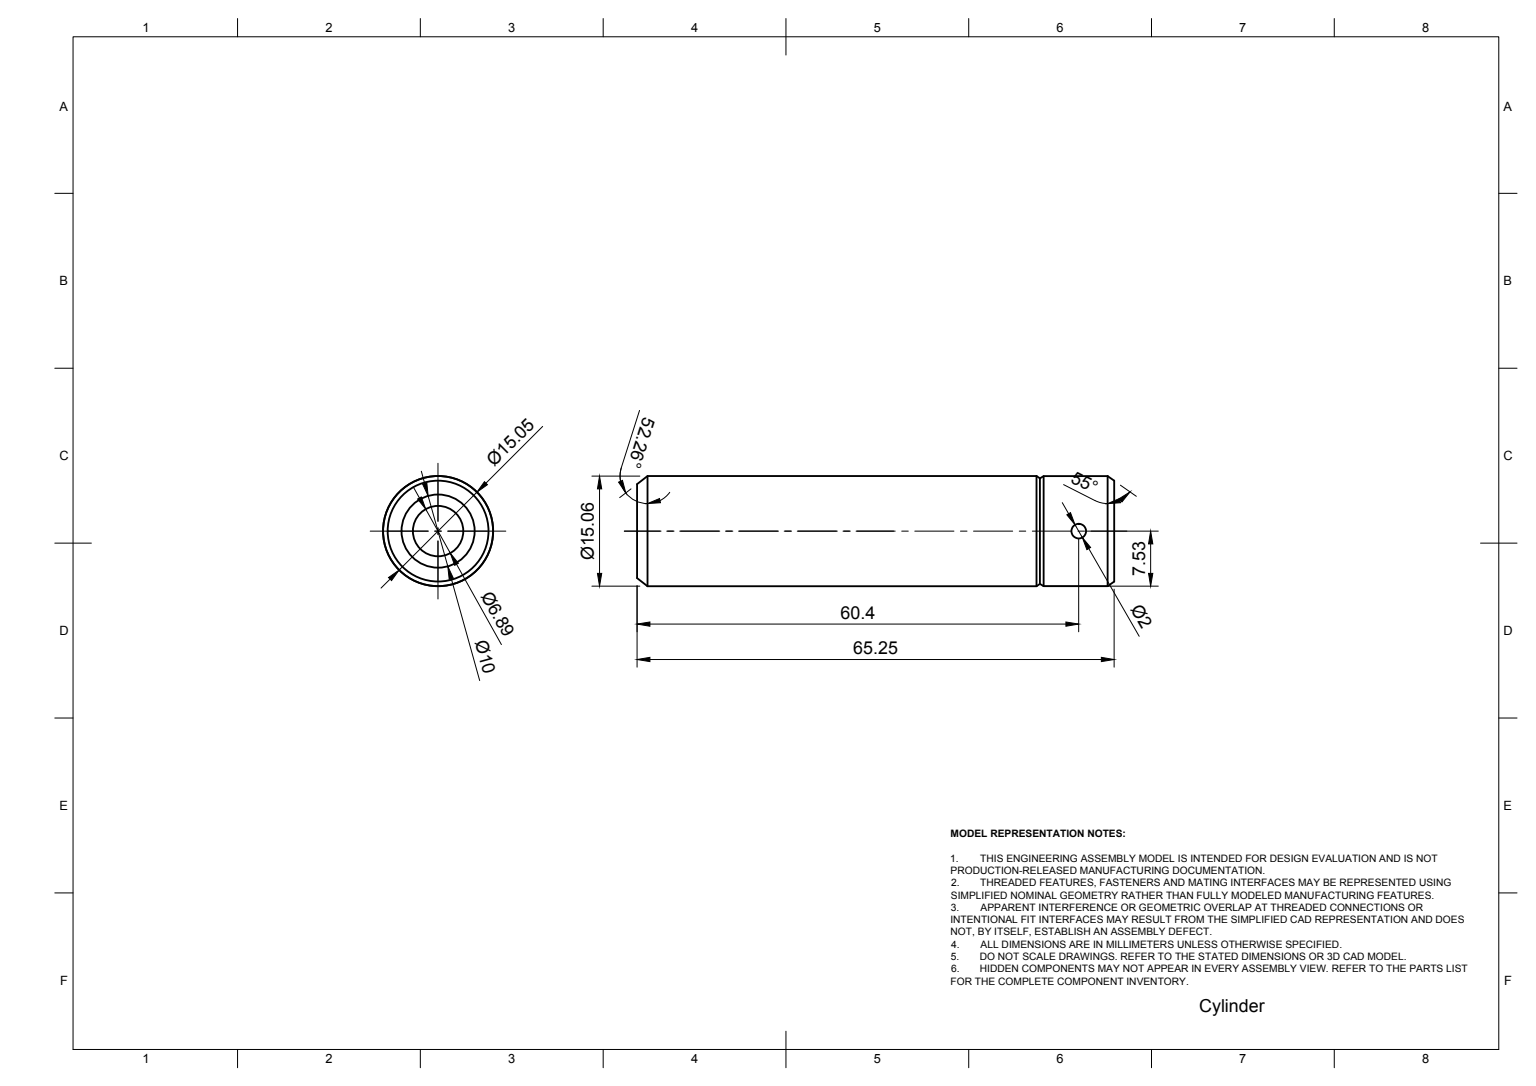
ISO-10303-21;
HEADER;
/* Generated by software containing ST-Developer
 * from STEP Tools, Inc. (www.steptools.com) 
 */

FILE_DESCRIPTION(
/* description */ (''),
/* implementation_level */ '2;1');

FILE_NAME(
/* name */ 'Cylinder.step',
/* time_stamp */ '2026-10-06T13:05:37-07:00',
/* author */ (''),
/* organization */ (''),
/* preprocessor_version */ 'ST-DEVELOPER v20.2',
/* originating_system */ 'Autodesk Translation Framework v15.15.0.0',
/* authorisation */ '');

FILE_SCHEMA (('AUTOMOTIVE_DESIGN { 1 0 10303 214 3 1 1 }'));
ENDSEC;

DATA;
#10=MECHANICAL_DESIGN_GEOMETRIC_PRESENTATION_REPRESENTATION('',(#136),#28055);
#116=SHAPE_REPRESENTATION_RELATIONSHIP('SRR','None',#28093,#126);
#126=ADVANCED_BREP_SHAPE_REPRESENTATION('',(#146),#28045);
#136=STYLED_ITEM('',(#28152),#146);
#146=MANIFOLD_SOLID_BREP('Body1',#3677);
#155=CONICAL_SURFACE('',#3808,7.20746054905241,0.610790367386849);
#156=CONICAL_SURFACE('',#3813,7.36529369971832,0.557210682142491);
#157=CONICAL_SURFACE('',#3815,7.36790580323689,0.610790367386849);
#158=CONICAL_SURFACE('',#3819,6.97561584944256,0.658634244892553);
#159=CONICAL_SURFACE('',#3821,6.41628586403442,0.000295609290232646);
#160=CONICAL_SURFACE('',#3825,6.40906719549494,0.00029560929023293);
#161=CONICAL_SURFACE('',#3833,6.40820475053297,0.000295609290233083);
#162=CONICAL_SURFACE('',#3837,6.40732538114918,0.000295609290232334);
#163=CONICAL_SURFACE('',#3841,6.40667124022599,0.000295609290231853);
#173=FACE_BOUND('',#588,.T.);
#174=FACE_BOUND('',#591,.T.);
#175=FACE_BOUND('',#600,.T.);
#176=FACE_BOUND('',#603,.T.);
#177=FACE_BOUND('',#610,.T.);
#178=FACE_BOUND('',#613,.T.);
#179=FACE_BOUND('',#615,.T.);
#180=FACE_BOUND('',#617,.T.);
#203=PLANE('',#3806);
#204=PLANE('',#3827);
#205=PLANE('',#3831);
#206=PLANE('',#3843);
#207=PLANE('',#3847);
#208=PLANE('',#3850);
#256=CIRCLE('',#3804,5.);
#257=CIRCLE('',#3805,5.);
#258=CIRCLE('',#3807,3.44589712386029);
#259=CIRCLE('',#3809,7.52312685038423);
#260=CIRCLE('',#3810,6.89179424772059);
#261=CIRCLE('',#3812,7.52312685038423);
#262=CIRCLE('',#3814,7.20746054905241);
#263=CIRCLE('',#3816,7.52835105742136);
#264=CIRCLE('',#3818,7.52835105742136);
#265=CIRCLE('',#3820,6.42288064146375);
#266=CIRCLE('',#3822,6.40969108660508);
#267=CIRCLE('',#3824,6.40969108660508);
#268=CIRCLE('',#3826,6.40881029802658);
#269=CIRCLE('',#3828,6.41550316824698);
#270=CIRCLE('',#3830,6.41550316824698);
#271=CIRCLE('',#3832,6.40853872070288);
#272=CIRCLE('',#3834,6.40787078036307);
#273=CIRCLE('',#3836,6.40787078036307);
#274=CIRCLE('',#3838,6.40706623219228);
#275=CIRCLE('',#3840,6.40706623219228);
#276=CIRCLE('',#3842,6.4065967297173);
#277=CIRCLE('',#3844,4.66385643997278);
#278=CIRCLE('',#3846,4.66385643997278);
#279=CIRCLE('',#3848,3.44589712386029);
#379=FACE_OUTER_BOUND('',#585,.T.);
#380=FACE_OUTER_BOUND('',#586,.T.);
#381=FACE_OUTER_BOUND('',#587,.T.);
#382=FACE_OUTER_BOUND('',#589,.T.);
#383=FACE_OUTER_BOUND('',#590,.T.);
#384=FACE_OUTER_BOUND('',#592,.T.);
#385=FACE_OUTER_BOUND('',#593,.T.);
#386=FACE_OUTER_BOUND('',#594,.T.);
#387=FACE_OUTER_BOUND('',#595,.T.);
#388=FACE_OUTER_BOUND('',#596,.T.);
#389=FACE_OUTER_BOUND('',#597,.T.);
#390=FACE_OUTER_BOUND('',#598,.T.);
#391=FACE_OUTER_BOUND('',#599,.T.);
#392=FACE_OUTER_BOUND('',#601,.T.);
#393=FACE_OUTER_BOUND('',#602,.T.);
#394=FACE_OUTER_BOUND('',#604,.T.);
#395=FACE_OUTER_BOUND('',#605,.T.);
#396=FACE_OUTER_BOUND('',#606,.T.);
#397=FACE_OUTER_BOUND('',#607,.T.);
#398=FACE_OUTER_BOUND('',#608,.T.);
#399=FACE_OUTER_BOUND('',#609,.T.);
#400=FACE_OUTER_BOUND('',#611,.T.);
#401=FACE_OUTER_BOUND('',#612,.T.);
#402=FACE_OUTER_BOUND('',#614,.T.);
#403=FACE_OUTER_BOUND('',#616,.T.);
#585=EDGE_LOOP('',(#2310,#2311,#2312,#2313,#2314,#2315));
#586=EDGE_LOOP('',(#2316,#2317,#2318,#2319));
#587=EDGE_LOOP('',(#2320));
#588=EDGE_LOOP('',(#2321));
#589=EDGE_LOOP('',(#2322,#2323,#2324,#2325));
#590=EDGE_LOOP('',(#2326,#2327,#2328,#2329));
#591=EDGE_LOOP('',(#2330,#2331));
#592=EDGE_LOOP('',(#2332,#2333,#2334,#2335));
#593=EDGE_LOOP('',(#2336,#2337,#2338,#2339));
#594=EDGE_LOOP('',(#2340,#2341,#2342,#2343));
#595=EDGE_LOOP('',(#2344,#2345,#2346,#2347));
#596=EDGE_LOOP('',(#2348,#2349,#2350,#2351));
#597=EDGE_LOOP('',(#2352,#2353,#2354,#2355));
#598=EDGE_LOOP('',(#2356,#2357,#2358,#2359));
#599=EDGE_LOOP('',(#2360));
#600=EDGE_LOOP('',(#2361));
#601=EDGE_LOOP('',(#2362,#2363,#2364,#2365));
#602=EDGE_LOOP('',(#2366));
#603=EDGE_LOOP('',(#2367));
#604=EDGE_LOOP('',(#2368,#2369,#2370,#2371));
#605=EDGE_LOOP('',(#2372,#2373,#2374,#2375));
#606=EDGE_LOOP('',(#2376,#2377,#2378,#2379));
#607=EDGE_LOOP('',(#2380,#2381,#2382,#2383));
#608=EDGE_LOOP('',(#2384,#2385,#2386,#2387));
#609=EDGE_LOOP('',(#2388));
#610=EDGE_LOOP('',(#2389));
#611=EDGE_LOOP('',(#2390,#2391,#2392,#2393));
#612=EDGE_LOOP('',(#2394));
#613=EDGE_LOOP('',(#2395));
#614=EDGE_LOOP('',(#2396,#2397,#2398,#2399));
#615=EDGE_LOOP('',(#2400,#2401));
#616=EDGE_LOOP('',(#2402));
#617=EDGE_LOOP('',(#2403));
#821=LINE('',#4942,#979);
#822=LINE('',#4984,#980);
#823=LINE('',#4993,#981);
#824=LINE('',#4998,#982);
#825=LINE('',#5001,#983);
#826=LINE('',#5006,#984);
#827=LINE('',#5010,#985);
#828=LINE('',#5013,#986);
#829=LINE('',#5018,#987);
#830=LINE('',#5022,#988);
#831=LINE('',#5026,#989);
#832=LINE('',#5033,#990);
#833=LINE('',#5040,#991);
#834=LINE('',#5044,#992);
#835=LINE('',#5048,#993);
#836=LINE('',#5052,#994);
#837=LINE('',#5056,#995);
#838=LINE('',#5063,#996);
#839=LINE('',#5068,#997);
#979=VECTOR('',#4120,0.999999999999999);
#980=VECTOR('',#4125,5.);
#981=VECTOR('',#4136,7.20746054905241);
#982=VECTOR('',#4143,7.52312685038423);
#983=VECTOR('',#4146,7.36529369971832);
#984=VECTOR('',#4153,7.36790580323689);
#985=VECTOR('',#4158,7.52835105742136);
#986=VECTOR('',#4161,6.97561584944256);
#987=VECTOR('',#4168,6.41628586403442);
#988=VECTOR('',#4173,6.40969108660508);
#989=VECTOR('',#4178,6.40906719549494);
#990=VECTOR('',#4187,6.41550316824698);
#991=VECTOR('',#4196,6.40820475053297);
#992=VECTOR('',#4201,6.40787078036307);
#993=VECTOR('',#4206,6.40732538114918);
#994=VECTOR('',#4211,6.40706623219228);
#995=VECTOR('',#4216,6.40667124022599);
#996=VECTOR('',#4225,4.66385643997278);
#997=VECTOR('',#4232,3.44589712386029);
#1137=B_SPLINE_CURVE_WITH_KNOTS('',3,(#4905,#4906,#4907,#4908,#4909,#4910,
#4911,#4912,#4913,#4914,#4915,#4916,#4917,#4918,#4919,#4920,#4921,#4922,
#4923,#4924,#4925,#4926,#4927,#4928,#4929,#4930),.UNSPECIFIED.,.F.,.F.,
(4,2,2,2,2,2,2,2,2,2,2,2,4),(-0.606481282784619,-0.568571286664201,-0.530661290543783,
-0.492761126316124,-0.454860962088464,-0.416960797860805,-0.379060633633146,
-0.341150637512728,-0.30324064139231,-0.265330645271891,-0.227420649151473,
-0.189520484923814,-0.151620320696155),.UNSPECIFIED.);
#1138=B_SPLINE_CURVE_WITH_KNOTS('',3,(#4931,#4932,#4933,#4934,#4935,#4936,
#4937,#4938,#4939,#4940),.UNSPECIFIED.,.F.,.F.,(4,2,2,2,4),(-0.151620320696155,
-0.113720156468496,-0.0758199922408364,-0.0379099961204182,0.),
 .UNSPECIFIED.);
#1139=B_SPLINE_CURVE_WITH_KNOTS('',3,(#4944,#4945,#4946,#4947,#4948,#4949,
#4950,#4951,#4952,#4953),.UNSPECIFIED.,.F.,.F.,(4,2,2,2,4),(0.,0.0377168406459521,
0.0754336812919042,0.113150118256495,0.150866555221085),.UNSPECIFIED.);
#1140=B_SPLINE_CURVE_WITH_KNOTS('',3,(#4954,#4955,#4956,#4957,#4958,#4959,
#4960,#4961,#4962,#4963,#4964,#4965,#4966,#4967,#4968,#4969,#4970,#4971,
#4972,#4973,#4974,#4975,#4976,#4977,#4978,#4979),.UNSPECIFIED.,.F.,.F.,
(4,2,2,2,2,2,2,2,2,2,2,2,4),(0.150866555221085,0.188582992185676,0.226299429150267,
0.264016269796219,0.301733110442171,0.339449951088123,0.377166791734075,
0.414883228698666,0.452599665663256,0.490316102627847,0.528032539592437,
0.565749380238389,0.603466220884342),.UNSPECIFIED.);
#1394=VERTEX_POINT('',#4903);
#1395=VERTEX_POINT('',#4904);
#1396=VERTEX_POINT('',#4941);
#1397=VERTEX_POINT('',#4943);
#1398=VERTEX_POINT('',#4981);
#1399=VERTEX_POINT('',#4983);
#1400=VERTEX_POINT('',#4987);
#1401=VERTEX_POINT('',#4990);
#1402=VERTEX_POINT('',#4992);
#1403=VERTEX_POINT('',#4996);
#1404=VERTEX_POINT('',#5000);
#1405=VERTEX_POINT('',#5004);
#1406=VERTEX_POINT('',#5008);
#1407=VERTEX_POINT('',#5012);
#1408=VERTEX_POINT('',#5016);
#1409=VERTEX_POINT('',#5020);
#1410=VERTEX_POINT('',#5024);
#1411=VERTEX_POINT('',#5028);
#1412=VERTEX_POINT('',#5031);
#1413=VERTEX_POINT('',#5035);
#1414=VERTEX_POINT('',#5038);
#1415=VERTEX_POINT('',#5042);
#1416=VERTEX_POINT('',#5046);
#1417=VERTEX_POINT('',#5050);
#1418=VERTEX_POINT('',#5054);
#1419=VERTEX_POINT('',#5058);
#1420=VERTEX_POINT('',#5061);
#1421=VERTEX_POINT('',#5065);
#1768=EDGE_CURVE('',#1394,#1395,#1137,.T.);
#1769=EDGE_CURVE('',#1395,#1394,#1138,.T.);
#1770=EDGE_CURVE('',#1395,#1396,#821,.T.);
#1771=EDGE_CURVE('',#1397,#1396,#1139,.T.);
#1772=EDGE_CURVE('',#1396,#1397,#1140,.T.);
#1773=EDGE_CURVE('',#1398,#1398,#256,.T.);
#1774=EDGE_CURVE('',#1398,#1399,#822,.T.);
#1775=EDGE_CURVE('',#1399,#1399,#257,.T.);
#1776=EDGE_CURVE('',#1400,#1400,#258,.T.);
#1777=EDGE_CURVE('',#1401,#1401,#259,.T.);
#1778=EDGE_CURVE('',#1401,#1402,#823,.T.);
#1779=EDGE_CURVE('',#1402,#1402,#260,.T.);
#1780=EDGE_CURVE('',#1403,#1403,#261,.T.);
#1781=EDGE_CURVE('',#1403,#1401,#824,.T.);
#1782=EDGE_CURVE('',#1403,#1404,#825,.T.);
#1783=EDGE_CURVE('',#1404,#1404,#262,.T.);
#1784=EDGE_CURVE('',#1405,#1405,#263,.T.);
#1785=EDGE_CURVE('',#1405,#1404,#826,.T.);
#1786=EDGE_CURVE('',#1406,#1406,#264,.T.);
#1787=EDGE_CURVE('',#1406,#1405,#827,.T.);
#1788=EDGE_CURVE('',#1406,#1407,#828,.T.);
#1789=EDGE_CURVE('',#1407,#1407,#265,.T.);
#1790=EDGE_CURVE('',#1408,#1408,#266,.T.);
#1791=EDGE_CURVE('',#1408,#1407,#829,.T.);
#1792=EDGE_CURVE('',#1409,#1409,#267,.T.);
#1793=EDGE_CURVE('',#1409,#1408,#830,.T.);
#1794=EDGE_CURVE('',#1410,#1410,#268,.T.);
#1795=EDGE_CURVE('',#1410,#1409,#831,.T.);
#1796=EDGE_CURVE('',#1411,#1411,#269,.T.);
#1797=EDGE_CURVE('',#1412,#1412,#270,.T.);
#1798=EDGE_CURVE('',#1412,#1411,#832,.T.);
#1799=EDGE_CURVE('',#1413,#1413,#271,.T.);
#1800=EDGE_CURVE('',#1414,#1414,#272,.T.);
#1801=EDGE_CURVE('',#1414,#1413,#833,.T.);
#1802=EDGE_CURVE('',#1415,#1415,#273,.T.);
#1803=EDGE_CURVE('',#1415,#1414,#834,.T.);
#1804=EDGE_CURVE('',#1416,#1416,#274,.T.);
#1805=EDGE_CURVE('',#1416,#1415,#835,.T.);
#1806=EDGE_CURVE('',#1417,#1417,#275,.T.);
#1807=EDGE_CURVE('',#1417,#1416,#836,.T.);
#1808=EDGE_CURVE('',#1418,#1418,#276,.T.);
#1809=EDGE_CURVE('',#1418,#1417,#837,.T.);
#1810=EDGE_CURVE('',#1419,#1419,#277,.T.);
#1811=EDGE_CURVE('',#1420,#1420,#278,.T.);
#1812=EDGE_CURVE('',#1420,#1419,#838,.T.);
#1813=EDGE_CURVE('',#1421,#1421,#279,.T.);
#1814=EDGE_CURVE('',#1400,#1421,#839,.T.);
#2310=ORIENTED_EDGE('',*,*,#1768,.F.);
#2311=ORIENTED_EDGE('',*,*,#1769,.F.);
#2312=ORIENTED_EDGE('',*,*,#1770,.T.);
#2313=ORIENTED_EDGE('',*,*,#1771,.F.);
#2314=ORIENTED_EDGE('',*,*,#1772,.F.);
#2315=ORIENTED_EDGE('',*,*,#1770,.F.);
#2316=ORIENTED_EDGE('',*,*,#1773,.F.);
#2317=ORIENTED_EDGE('',*,*,#1774,.T.);
#2318=ORIENTED_EDGE('',*,*,#1775,.T.);
#2319=ORIENTED_EDGE('',*,*,#1774,.F.);
#2320=ORIENTED_EDGE('',*,*,#1775,.F.);
#2321=ORIENTED_EDGE('',*,*,#1776,.T.);
#2322=ORIENTED_EDGE('',*,*,#1777,.F.);
#2323=ORIENTED_EDGE('',*,*,#1778,.T.);
#2324=ORIENTED_EDGE('',*,*,#1779,.T.);
#2325=ORIENTED_EDGE('',*,*,#1778,.F.);
#2326=ORIENTED_EDGE('',*,*,#1780,.F.);
#2327=ORIENTED_EDGE('',*,*,#1781,.T.);
#2328=ORIENTED_EDGE('',*,*,#1777,.T.);
#2329=ORIENTED_EDGE('',*,*,#1781,.F.);
#2330=ORIENTED_EDGE('',*,*,#1771,.T.);
#2331=ORIENTED_EDGE('',*,*,#1772,.T.);
#2332=ORIENTED_EDGE('',*,*,#1780,.T.);
#2333=ORIENTED_EDGE('',*,*,#1782,.T.);
#2334=ORIENTED_EDGE('',*,*,#1783,.F.);
#2335=ORIENTED_EDGE('',*,*,#1782,.F.);
#2336=ORIENTED_EDGE('',*,*,#1784,.F.);
#2337=ORIENTED_EDGE('',*,*,#1785,.T.);
#2338=ORIENTED_EDGE('',*,*,#1783,.T.);
#2339=ORIENTED_EDGE('',*,*,#1785,.F.);
#2340=ORIENTED_EDGE('',*,*,#1786,.F.);
#2341=ORIENTED_EDGE('',*,*,#1787,.T.);
#2342=ORIENTED_EDGE('',*,*,#1784,.T.);
#2343=ORIENTED_EDGE('',*,*,#1787,.F.);
#2344=ORIENTED_EDGE('',*,*,#1786,.T.);
#2345=ORIENTED_EDGE('',*,*,#1788,.T.);
#2346=ORIENTED_EDGE('',*,*,#1789,.F.);
#2347=ORIENTED_EDGE('',*,*,#1788,.F.);
#2348=ORIENTED_EDGE('',*,*,#1790,.F.);
#2349=ORIENTED_EDGE('',*,*,#1791,.T.);
#2350=ORIENTED_EDGE('',*,*,#1789,.T.);
#2351=ORIENTED_EDGE('',*,*,#1791,.F.);
#2352=ORIENTED_EDGE('',*,*,#1792,.F.);
#2353=ORIENTED_EDGE('',*,*,#1793,.T.);
#2354=ORIENTED_EDGE('',*,*,#1790,.T.);
#2355=ORIENTED_EDGE('',*,*,#1793,.F.);
#2356=ORIENTED_EDGE('',*,*,#1794,.F.);
#2357=ORIENTED_EDGE('',*,*,#1795,.T.);
#2358=ORIENTED_EDGE('',*,*,#1792,.T.);
#2359=ORIENTED_EDGE('',*,*,#1795,.F.);
#2360=ORIENTED_EDGE('',*,*,#1796,.F.);
#2361=ORIENTED_EDGE('',*,*,#1794,.T.);
#2362=ORIENTED_EDGE('',*,*,#1797,.F.);
#2363=ORIENTED_EDGE('',*,*,#1798,.T.);
#2364=ORIENTED_EDGE('',*,*,#1796,.T.);
#2365=ORIENTED_EDGE('',*,*,#1798,.F.);
#2366=ORIENTED_EDGE('',*,*,#1797,.T.);
#2367=ORIENTED_EDGE('',*,*,#1799,.F.);
#2368=ORIENTED_EDGE('',*,*,#1800,.F.);
#2369=ORIENTED_EDGE('',*,*,#1801,.T.);
#2370=ORIENTED_EDGE('',*,*,#1799,.T.);
#2371=ORIENTED_EDGE('',*,*,#1801,.F.);
#2372=ORIENTED_EDGE('',*,*,#1802,.F.);
#2373=ORIENTED_EDGE('',*,*,#1803,.T.);
#2374=ORIENTED_EDGE('',*,*,#1800,.T.);
#2375=ORIENTED_EDGE('',*,*,#1803,.F.);
#2376=ORIENTED_EDGE('',*,*,#1804,.F.);
#2377=ORIENTED_EDGE('',*,*,#1805,.T.);
#2378=ORIENTED_EDGE('',*,*,#1802,.T.);
#2379=ORIENTED_EDGE('',*,*,#1805,.F.);
#2380=ORIENTED_EDGE('',*,*,#1806,.F.);
#2381=ORIENTED_EDGE('',*,*,#1807,.T.);
#2382=ORIENTED_EDGE('',*,*,#1804,.T.);
#2383=ORIENTED_EDGE('',*,*,#1807,.F.);
#2384=ORIENTED_EDGE('',*,*,#1808,.F.);
#2385=ORIENTED_EDGE('',*,*,#1809,.T.);
#2386=ORIENTED_EDGE('',*,*,#1806,.T.);
#2387=ORIENTED_EDGE('',*,*,#1809,.F.);
#2388=ORIENTED_EDGE('',*,*,#1808,.T.);
#2389=ORIENTED_EDGE('',*,*,#1810,.F.);
#2390=ORIENTED_EDGE('',*,*,#1811,.F.);
#2391=ORIENTED_EDGE('',*,*,#1812,.T.);
#2392=ORIENTED_EDGE('',*,*,#1810,.T.);
#2393=ORIENTED_EDGE('',*,*,#1812,.F.);
#2394=ORIENTED_EDGE('',*,*,#1811,.T.);
#2395=ORIENTED_EDGE('',*,*,#1813,.F.);
#2396=ORIENTED_EDGE('',*,*,#1776,.F.);
#2397=ORIENTED_EDGE('',*,*,#1814,.T.);
#2398=ORIENTED_EDGE('',*,*,#1813,.T.);
#2399=ORIENTED_EDGE('',*,*,#1814,.F.);
#2400=ORIENTED_EDGE('',*,*,#1768,.T.);
#2401=ORIENTED_EDGE('',*,*,#1769,.T.);
#2402=ORIENTED_EDGE('',*,*,#1779,.F.);
#2403=ORIENTED_EDGE('',*,*,#1773,.T.);
#3394=CYLINDRICAL_SURFACE('',#3802,0.999999999999999);
#3395=CYLINDRICAL_SURFACE('',#3803,5.);
#3396=CYLINDRICAL_SURFACE('',#3811,7.52312685038423);
#3397=CYLINDRICAL_SURFACE('',#3817,7.52835105742136);
#3398=CYLINDRICAL_SURFACE('',#3823,6.40969108660508);
#3399=CYLINDRICAL_SURFACE('',#3829,6.41550316824698);
#3400=CYLINDRICAL_SURFACE('',#3835,6.40787078036307);
#3401=CYLINDRICAL_SURFACE('',#3839,6.40706623219228);
#3402=CYLINDRICAL_SURFACE('',#3845,4.66385643997278);
#3403=CYLINDRICAL_SURFACE('',#3849,3.44589712386029);
#3471=ADVANCED_FACE('',(#379),#3394,.F.);
#3472=ADVANCED_FACE('',(#380),#3395,.F.);
#3473=ADVANCED_FACE('',(#381,#173),#203,.T.);
#3474=ADVANCED_FACE('',(#382),#155,.T.);
#3475=ADVANCED_FACE('',(#383,#174),#3396,.T.);
#3476=ADVANCED_FACE('',(#384),#156,.T.);
#3477=ADVANCED_FACE('',(#385),#157,.T.);
#3478=ADVANCED_FACE('',(#386),#3397,.T.);
#3479=ADVANCED_FACE('',(#387),#158,.T.);
#3480=ADVANCED_FACE('',(#388),#159,.F.);
#3481=ADVANCED_FACE('',(#389),#3398,.F.);
#3482=ADVANCED_FACE('',(#390),#160,.F.);
#3483=ADVANCED_FACE('',(#391,#175),#204,.T.);
#3484=ADVANCED_FACE('',(#392),#3399,.F.);
#3485=ADVANCED_FACE('',(#393,#176),#205,.T.);
#3486=ADVANCED_FACE('',(#394),#161,.F.);
#3487=ADVANCED_FACE('',(#395),#3400,.F.);
#3488=ADVANCED_FACE('',(#396),#162,.F.);
#3489=ADVANCED_FACE('',(#397),#3401,.F.);
#3490=ADVANCED_FACE('',(#398),#163,.F.);
#3491=ADVANCED_FACE('',(#399,#177),#206,.T.);
#3492=ADVANCED_FACE('',(#400),#3402,.F.);
#3493=ADVANCED_FACE('',(#401,#178),#207,.T.);
#3494=ADVANCED_FACE('',(#402,#179),#3403,.F.);
#3495=ADVANCED_FACE('',(#403,#180),#208,.T.);
#3677=CLOSED_SHELL('',(#3471,#3472,#3473,#3474,#3475,#3476,#3477,#3478,
#3479,#3480,#3481,#3482,#3483,#3484,#3485,#3486,#3487,#3488,#3489,#3490,
#3491,#3492,#3493,#3494,#3495));
#3801=AXIS2_PLACEMENT_3D('',#4901,#4116,#4117);
#3802=AXIS2_PLACEMENT_3D('',#4902,#4118,#4119);
#3803=AXIS2_PLACEMENT_3D('',#4980,#4121,#4122);
#3804=AXIS2_PLACEMENT_3D('',#4982,#4123,#4124);
#3805=AXIS2_PLACEMENT_3D('',#4985,#4126,#4127);
#3806=AXIS2_PLACEMENT_3D('',#4986,#4128,#4129);
#3807=AXIS2_PLACEMENT_3D('',#4988,#4130,#4131);
#3808=AXIS2_PLACEMENT_3D('',#4989,#4132,#4133);
#3809=AXIS2_PLACEMENT_3D('',#4991,#4134,#4135);
#3810=AXIS2_PLACEMENT_3D('',#4994,#4137,#4138);
#3811=AXIS2_PLACEMENT_3D('',#4995,#4139,#4140);
#3812=AXIS2_PLACEMENT_3D('',#4997,#4141,#4142);
#3813=AXIS2_PLACEMENT_3D('',#4999,#4144,#4145);
#3814=AXIS2_PLACEMENT_3D('',#5002,#4147,#4148);
#3815=AXIS2_PLACEMENT_3D('',#5003,#4149,#4150);
#3816=AXIS2_PLACEMENT_3D('',#5005,#4151,#4152);
#3817=AXIS2_PLACEMENT_3D('',#5007,#4154,#4155);
#3818=AXIS2_PLACEMENT_3D('',#5009,#4156,#4157);
#3819=AXIS2_PLACEMENT_3D('',#5011,#4159,#4160);
#3820=AXIS2_PLACEMENT_3D('',#5014,#4162,#4163);
#3821=AXIS2_PLACEMENT_3D('',#5015,#4164,#4165);
#3822=AXIS2_PLACEMENT_3D('',#5017,#4166,#4167);
#3823=AXIS2_PLACEMENT_3D('',#5019,#4169,#4170);
#3824=AXIS2_PLACEMENT_3D('',#5021,#4171,#4172);
#3825=AXIS2_PLACEMENT_3D('',#5023,#4174,#4175);
#3826=AXIS2_PLACEMENT_3D('',#5025,#4176,#4177);
#3827=AXIS2_PLACEMENT_3D('',#5027,#4179,#4180);
#3828=AXIS2_PLACEMENT_3D('',#5029,#4181,#4182);
#3829=AXIS2_PLACEMENT_3D('',#5030,#4183,#4184);
#3830=AXIS2_PLACEMENT_3D('',#5032,#4185,#4186);
#3831=AXIS2_PLACEMENT_3D('',#5034,#4188,#4189);
#3832=AXIS2_PLACEMENT_3D('',#5036,#4190,#4191);
#3833=AXIS2_PLACEMENT_3D('',#5037,#4192,#4193);
#3834=AXIS2_PLACEMENT_3D('',#5039,#4194,#4195);
#3835=AXIS2_PLACEMENT_3D('',#5041,#4197,#4198);
#3836=AXIS2_PLACEMENT_3D('',#5043,#4199,#4200);
#3837=AXIS2_PLACEMENT_3D('',#5045,#4202,#4203);
#3838=AXIS2_PLACEMENT_3D('',#5047,#4204,#4205);
#3839=AXIS2_PLACEMENT_3D('',#5049,#4207,#4208);
#3840=AXIS2_PLACEMENT_3D('',#5051,#4209,#4210);
#3841=AXIS2_PLACEMENT_3D('',#5053,#4212,#4213);
#3842=AXIS2_PLACEMENT_3D('',#5055,#4214,#4215);
#3843=AXIS2_PLACEMENT_3D('',#5057,#4217,#4218);
#3844=AXIS2_PLACEMENT_3D('',#5059,#4219,#4220);
#3845=AXIS2_PLACEMENT_3D('',#5060,#4221,#4222);
#3846=AXIS2_PLACEMENT_3D('',#5062,#4223,#4224);
#3847=AXIS2_PLACEMENT_3D('',#5064,#4226,#4227);
#3848=AXIS2_PLACEMENT_3D('',#5066,#4228,#4229);
#3849=AXIS2_PLACEMENT_3D('',#5067,#4230,#4231);
#3850=AXIS2_PLACEMENT_3D('',#5069,#4233,#4234);
#4116=DIRECTION('axis',(0.,0.,1.));
#4117=DIRECTION('refdir',(1.,0.,0.));
#4118=DIRECTION('center_axis',(0.,1.,0.));
#4119=DIRECTION('ref_axis',(1.,0.,0.));
#4120=DIRECTION('',(0.,1.,0.));
#4121=DIRECTION('center_axis',(1.,0.,0.));
#4122=DIRECTION('ref_axis',(0.,-1.,0.));
#4123=DIRECTION('center_axis',(1.,0.,0.));
#4124=DIRECTION('ref_axis',(0.,-1.,0.));
#4125=DIRECTION('',(1.,0.,0.));
#4126=DIRECTION('center_axis',(1.,0.,0.));
#4127=DIRECTION('ref_axis',(0.,-1.,0.));
#4128=DIRECTION('center_axis',(-1.,0.,0.));
#4129=DIRECTION('ref_axis',(0.,-1.,0.));
#4130=DIRECTION('center_axis',(1.,0.,0.));
#4131=DIRECTION('ref_axis',(0.,0.,-1.));
#4132=DIRECTION('center_axis',(1.,0.,0.));
#4133=DIRECTION('ref_axis',(0.,0.,-1.));
#4134=DIRECTION('center_axis',(1.,0.,0.));
#4135=DIRECTION('ref_axis',(0.,0.,-1.));
#4136=DIRECTION('',(-0.819194986126072,7.02353436578877E-17,-0.573515104165448));
#4137=DIRECTION('center_axis',(1.,0.,0.));
#4138=DIRECTION('ref_axis',(0.,0.,-1.));
#4139=DIRECTION('center_axis',(1.,0.,0.));
#4140=DIRECTION('ref_axis',(0.,0.,-1.));
#4141=DIRECTION('center_axis',(1.,0.,0.));
#4142=DIRECTION('ref_axis',(0.,0.,-1.));
#4143=DIRECTION('',(-1.,0.,0.));
#4144=DIRECTION('center_axis',(-1.,0.,0.));
#4145=DIRECTION('ref_axis',(0.,0.,-1.));
#4146=DIRECTION('',(0.848733460294827,-6.47618786727041E-17,-0.528820870783264));
#4147=DIRECTION('center_axis',(1.,0.,0.));
#4148=DIRECTION('ref_axis',(0.,0.,-1.));
#4149=DIRECTION('center_axis',(1.,0.,0.));
#4150=DIRECTION('ref_axis',(0.,0.,-1.));
#4151=DIRECTION('center_axis',(1.,0.,0.));
#4152=DIRECTION('ref_axis',(0.,0.,-1.));
#4153=DIRECTION('',(-0.819194986126072,7.02353436578877E-17,-0.573515104165448));
#4154=DIRECTION('center_axis',(1.,0.,0.));
#4155=DIRECTION('ref_axis',(0.,0.,-1.));
#4156=DIRECTION('center_axis',(1.,0.,0.));
#4157=DIRECTION('ref_axis',(0.,0.,-1.));
#4158=DIRECTION('',(-1.,0.,0.));
#4159=DIRECTION('center_axis',(-1.,0.,0.));
#4160=DIRECTION('ref_axis',(0.,0.,-1.));
#4161=DIRECTION('',(0.790828861928077,-7.49529574979538E-17,-0.612037344564482));
#4162=DIRECTION('center_axis',(1.,0.,0.));
#4163=DIRECTION('ref_axis',(0.,0.,-1.));
#4164=DIRECTION('center_axis',(1.,0.,0.));
#4165=DIRECTION('ref_axis',(0.,0.,-1.));
#4166=DIRECTION('center_axis',(1.,0.,0.));
#4167=DIRECTION('ref_axis',(0.,0.,-1.));
#4168=DIRECTION('',(0.999999956307574,-3.62016965809164E-20,0.00029560928592735));
#4169=DIRECTION('center_axis',(1.,0.,0.));
#4170=DIRECTION('ref_axis',(0.,0.,-1.));
#4171=DIRECTION('center_axis',(1.,0.,0.));
#4172=DIRECTION('ref_axis',(0.,0.,-1.));
#4173=DIRECTION('',(1.,0.,0.));
#4174=DIRECTION('center_axis',(1.,0.,0.));
#4175=DIRECTION('ref_axis',(0.,0.,-1.));
#4176=DIRECTION('center_axis',(1.,0.,0.));
#4177=DIRECTION('ref_axis',(0.,0.,-1.));
#4178=DIRECTION('',(0.999999956307574,-3.62016965809512E-20,0.000295609285927634));
#4179=DIRECTION('center_axis',(-1.,0.,0.));
#4180=DIRECTION('ref_axis',(0.,0.,1.));
#4181=DIRECTION('center_axis',(1.,0.,0.));
#4182=DIRECTION('ref_axis',(0.,0.,-1.));
#4183=DIRECTION('center_axis',(1.,0.,0.));
#4184=DIRECTION('ref_axis',(0.,0.,-1.));
#4185=DIRECTION('center_axis',(1.,0.,0.));
#4186=DIRECTION('ref_axis',(0.,0.,-1.));
#4187=DIRECTION('',(1.,0.,0.));
#4188=DIRECTION('center_axis',(1.,0.,0.));
#4189=DIRECTION('ref_axis',(0.,0.,-1.));
#4190=DIRECTION('center_axis',(1.,0.,0.));
#4191=DIRECTION('ref_axis',(0.,0.,-1.));
#4192=DIRECTION('center_axis',(1.,0.,0.));
#4193=DIRECTION('ref_axis',(0.,0.,-1.));
#4194=DIRECTION('center_axis',(1.,0.,0.));
#4195=DIRECTION('ref_axis',(0.,0.,-1.));
#4196=DIRECTION('',(0.999999956307574,-3.62016965809699E-20,0.000295609285927787));
#4197=DIRECTION('center_axis',(1.,0.,0.));
#4198=DIRECTION('ref_axis',(0.,0.,-1.));
#4199=DIRECTION('center_axis',(1.,0.,0.));
#4200=DIRECTION('ref_axis',(0.,0.,-1.));
#4201=DIRECTION('',(1.,0.,0.));
#4202=DIRECTION('center_axis',(1.,0.,0.));
#4203=DIRECTION('ref_axis',(0.,0.,-1.));
#4204=DIRECTION('center_axis',(1.,0.,0.));
#4205=DIRECTION('ref_axis',(0.,0.,-1.));
#4206=DIRECTION('',(0.999999956307574,-3.62016965808782E-20,0.000295609285927038));
#4207=DIRECTION('center_axis',(1.,0.,0.));
#4208=DIRECTION('ref_axis',(0.,0.,-1.));
#4209=DIRECTION('center_axis',(1.,0.,0.));
#4210=DIRECTION('ref_axis',(0.,0.,-1.));
#4211=DIRECTION('',(1.,0.,0.));
#4212=DIRECTION('center_axis',(1.,0.,0.));
#4213=DIRECTION('ref_axis',(0.,0.,-1.));
#4214=DIRECTION('center_axis',(1.,0.,0.));
#4215=DIRECTION('ref_axis',(0.,0.,-1.));
#4216=DIRECTION('',(0.999999956307574,-3.62016965808193E-20,0.000295609285926557));
#4217=DIRECTION('center_axis',(1.,0.,0.));
#4218=DIRECTION('ref_axis',(0.,0.,-1.));
#4219=DIRECTION('center_axis',(1.,0.,0.));
#4220=DIRECTION('ref_axis',(0.,0.,-1.));
#4221=DIRECTION('center_axis',(1.,0.,0.));
#4222=DIRECTION('ref_axis',(0.,0.,-1.));
#4223=DIRECTION('center_axis',(1.,0.,0.));
#4224=DIRECTION('ref_axis',(0.,0.,-1.));
#4225=DIRECTION('',(1.,0.,0.));
#4226=DIRECTION('center_axis',(1.,0.,0.));
#4227=DIRECTION('ref_axis',(0.,0.,-1.));
#4228=DIRECTION('center_axis',(1.,0.,0.));
#4229=DIRECTION('ref_axis',(0.,0.,-1.));
#4230=DIRECTION('center_axis',(1.,0.,0.));
#4231=DIRECTION('ref_axis',(0.,0.,-1.));
#4232=DIRECTION('',(1.,0.,0.));
#4233=DIRECTION('center_axis',(-1.,0.,0.));
#4234=DIRECTION('ref_axis',(0.,0.,1.));
#4901=CARTESIAN_POINT('',(0.,0.,0.));
#4902=CARTESIAN_POINT('Origin',(15.8714473032184,0.,0.));
#4903=CARTESIAN_POINT('',(15.8714473032184,3.29760625124175,0.999999999999998));
#4904=CARTESIAN_POINT('',(14.8714473032184,3.44589712386029,-6.01983033610089E-17));
#4905=CARTESIAN_POINT('Ctrl Pts',(15.8714473032184,3.29760625124174,0.999999999999999));
#4906=CARTESIAN_POINT('Ctrl Pts',(15.9978139569531,3.29760625124174,0.999999999999999));
#4907=CARTESIAN_POINT('Ctrl Pts',(16.132068844028,3.30562953237115,0.974596096350375));
#4908=CARTESIAN_POINT('Ctrl Pts',(16.3782103010389,3.33407731229027,0.872325929581351));
#4909=CARTESIAN_POINT('Ctrl Pts',(16.4901654582252,3.3540348875684,0.795495407366277));
#4910=CARTESIAN_POINT('Ctrl Pts',(16.6669197871454,3.39109395594973,0.618741078446085));
#4911=CARTESIAN_POINT('Ctrl Pts',(16.7437680872924,3.41067812574963,0.506776556958312));
#4912=CARTESIAN_POINT('Ctrl Pts',(16.8460513462857,3.43826042485992,0.26060123975522));
#4913=CARTESIAN_POINT('Ctrl Pts',(16.8714473032184,3.44589712386029,0.126333880758864));
#4914=CARTESIAN_POINT('Ctrl Pts',(16.8714473032184,3.44589712386029,-0.126333880758864));
#4915=CARTESIAN_POINT('Ctrl Pts',(16.8460513462857,3.43826042485992,-0.260601239755222));
#4916=CARTESIAN_POINT('Ctrl Pts',(16.7437680872924,3.41067812574963,-0.506776556958312));
#4917=CARTESIAN_POINT('Ctrl Pts',(16.6669197871454,3.39109395594973,-0.618741078446085));
#4918=CARTESIAN_POINT('Ctrl Pts',(16.4901654582252,3.3540348875684,-0.795495407366277));
#4919=CARTESIAN_POINT('Ctrl Pts',(16.3782103010389,3.33407731229027,-0.872325929581349));
#4920=CARTESIAN_POINT('Ctrl Pts',(16.132068844028,3.30562953237115,-0.974596096350375));
#4921=CARTESIAN_POINT('Ctrl Pts',(15.9978139569531,3.29760625124174,-0.999999999999999));
#4922=CARTESIAN_POINT('Ctrl Pts',(15.7450806494837,3.29760625124174,-0.999999999999999));
#4923=CARTESIAN_POINT('Ctrl Pts',(15.6108257624088,3.30562953237115,-0.974596096350376));
#4924=CARTESIAN_POINT('Ctrl Pts',(15.3646843053979,3.33407731229027,-0.872325929581351));
#4925=CARTESIAN_POINT('Ctrl Pts',(15.2527291482116,3.3540348875684,-0.795495407366277));
#4926=CARTESIAN_POINT('Ctrl Pts',(15.0759748192914,3.39109395594973,-0.618741078446085));
#4927=CARTESIAN_POINT('Ctrl Pts',(14.9991265191444,3.41067812574963,-0.506776556958314));
#4928=CARTESIAN_POINT('Ctrl Pts',(14.8968432601511,3.43826042485992,-0.260601239755224));
#4929=CARTESIAN_POINT('Ctrl Pts',(14.8714473032184,3.44589712386029,-0.126333880758864));
#4930=CARTESIAN_POINT('Ctrl Pts',(14.8714473032184,3.44589712386029,-2.42861286636753E-16));
#4931=CARTESIAN_POINT('Ctrl Pts',(14.8714473032184,3.44589712386029,-1.38777878078145E-16));
#4932=CARTESIAN_POINT('Ctrl Pts',(14.8714473032184,3.44589712386029,0.126333880758864));
#4933=CARTESIAN_POINT('Ctrl Pts',(14.8968432601511,3.43826042485992,0.260601239755221));
#4934=CARTESIAN_POINT('Ctrl Pts',(14.9991265191444,3.41067812574963,0.506776556958312));
#4935=CARTESIAN_POINT('Ctrl Pts',(15.0759748192914,3.39109395594973,0.618741078446085));
#4936=CARTESIAN_POINT('Ctrl Pts',(15.2527291482116,3.3540348875684,0.795495407366277));
#4937=CARTESIAN_POINT('Ctrl Pts',(15.3646843053979,3.33407731229027,0.872325929581349));
#4938=CARTESIAN_POINT('Ctrl Pts',(15.6108257624088,3.30562953237115,0.974596096350375));
#4939=CARTESIAN_POINT('Ctrl Pts',(15.7450806494837,3.29760625124174,0.999999999999999));
#4940=CARTESIAN_POINT('Ctrl Pts',(15.8714473032184,3.29760625124174,0.999999999999999));
#4941=CARTESIAN_POINT('',(14.8714473032184,7.52312685038423,1.22464679914735E-16));
#4942=CARTESIAN_POINT('',(14.8714473032184,0.,1.22464679914735E-16));
#4943=CARTESIAN_POINT('',(15.8714473032184,7.45636892910833,0.999999999999999));
#4944=CARTESIAN_POINT('Ctrl Pts',(15.8714473032184,7.45636892910833,0.999999999999999));
#4945=CARTESIAN_POINT('Ctrl Pts',(15.7457245010652,7.45636892910833,0.999999999999999));
#4946=CARTESIAN_POINT('Ctrl Pts',(15.6117245964979,7.45987689127736,0.974843764196788));
#4947=CARTESIAN_POINT('Ctrl Pts',(15.3653900481838,7.47250970222183,0.872744136330349));
#4948=CARTESIAN_POINT('Ctrl Pts',(15.2530425360435,7.48144799782428,0.795808795198177));
#4949=CARTESIAN_POINT('Ctrl Pts',(15.0756394573932,7.49819644864561,0.618405716547907));
#4950=CARTESIAN_POINT('Ctrl Pts',(14.9987033720303,7.50710016352641,0.506057792670463));
#4951=CARTESIAN_POINT('Ctrl Pts',(14.8966032000273,7.51965370990447,0.259721846141313));
#4952=CARTESIAN_POINT('Ctrl Pts',(14.8714473032184,7.52312685038423,0.125721456548635));
#4953=CARTESIAN_POINT('Ctrl Pts',(14.8714473032184,7.52312685038423,-1.04083408558608E-16));
#4954=CARTESIAN_POINT('Ctrl Pts',(14.8714473032184,7.52312685038423,-2.08166817117217E-16));
#4955=CARTESIAN_POINT('Ctrl Pts',(14.8714473032184,7.52312685038423,-0.125721456548636));
#4956=CARTESIAN_POINT('Ctrl Pts',(14.8966032000273,7.51965370990447,-0.259721846141313));
#4957=CARTESIAN_POINT('Ctrl Pts',(14.9987033720303,7.50710016352641,-0.506057792670463));
#4958=CARTESIAN_POINT('Ctrl Pts',(15.0756394573932,7.49819644864561,-0.618405716547907));
#4959=CARTESIAN_POINT('Ctrl Pts',(15.2530425360435,7.48144799782428,-0.795808795198177));
#4960=CARTESIAN_POINT('Ctrl Pts',(15.3653900481838,7.47250970222183,-0.872744136330348));
#4961=CARTESIAN_POINT('Ctrl Pts',(15.6117245964979,7.45987689127736,-0.974843764196788));
#4962=CARTESIAN_POINT('Ctrl Pts',(15.7457245010652,7.45636892910833,-0.999999999999999));
#4963=CARTESIAN_POINT('Ctrl Pts',(15.9971701053716,7.45636892910833,-0.999999999999999));
#4964=CARTESIAN_POINT('Ctrl Pts',(16.1311700099389,7.45987689127736,-0.974843764196788));
#4965=CARTESIAN_POINT('Ctrl Pts',(16.377504558253,7.47250970222183,-0.872744136330349));
#4966=CARTESIAN_POINT('Ctrl Pts',(16.4898520703933,7.48144799782428,-0.795808795198177));
#4967=CARTESIAN_POINT('Ctrl Pts',(16.6672551490436,7.49819644864561,-0.618405716547907));
#4968=CARTESIAN_POINT('Ctrl Pts',(16.7441912344065,7.50710016352641,-0.506057792670463));
#4969=CARTESIAN_POINT('Ctrl Pts',(16.8462914064095,7.51965370990447,-0.259721846141313));
#4970=CARTESIAN_POINT('Ctrl Pts',(16.8714473032184,7.52312685038423,-0.125721456548635));
#4971=CARTESIAN_POINT('Ctrl Pts',(16.8714473032184,7.52312685038423,0.125721456548635));
#4972=CARTESIAN_POINT('Ctrl Pts',(16.8462914064095,7.51965370990447,0.259721846141313));
#4973=CARTESIAN_POINT('Ctrl Pts',(16.7441912344065,7.50710016352641,0.506057792670463));
#4974=CARTESIAN_POINT('Ctrl Pts',(16.6672551490436,7.49819644864561,0.618405716547907));
#4975=CARTESIAN_POINT('Ctrl Pts',(16.4898520703933,7.48144799782428,0.795808795198176));
#4976=CARTESIAN_POINT('Ctrl Pts',(16.377504558253,7.47250970222183,0.872744136330349));
#4977=CARTESIAN_POINT('Ctrl Pts',(16.1311700099389,7.45987689127736,0.974843764196788));
#4978=CARTESIAN_POINT('Ctrl Pts',(15.9971701053716,7.45636892910833,0.999999999999999));
#4979=CARTESIAN_POINT('Ctrl Pts',(15.8714473032184,7.45636892910833,0.999999999999999));
#4980=CARTESIAN_POINT('Origin',(11.0238490761438,0.,0.));
#4981=CARTESIAN_POINT('',(11.0238490761438,5.,-6.12323399573677E-16));
#4982=CARTESIAN_POINT('Origin',(11.0238490761438,0.,0.));
#4983=CARTESIAN_POINT('',(12.0767011645438,5.,-6.12323399573677E-16));
#4984=CARTESIAN_POINT('',(11.0238490761438,5.,6.12323399573677E-16));
#4985=CARTESIAN_POINT('Origin',(12.0767011645438,0.,0.));
#4986=CARTESIAN_POINT('Origin',(12.0767011645438,0.,0.));
#4987=CARTESIAN_POINT('',(12.076701164516,-4.22000688292658E-16,3.44589712386029));
#4988=CARTESIAN_POINT('Origin',(12.076701164516,0.,0.));
#4989=CARTESIAN_POINT('Origin',(11.474739121518,0.,0.));
#4990=CARTESIAN_POINT('',(11.9256291668923,-9.21317321690256E-16,7.52312685038423));
#4991=CARTESIAN_POINT('Origin',(11.9256291668923,0.,0.));
#4992=CARTESIAN_POINT('',(11.0238490761438,-8.44001376585316E-16,6.89179424772059));
#4993=CARTESIAN_POINT('',(11.474739121518,-8.82659349137786E-16,7.20746054905241));
#4994=CARTESIAN_POINT('Origin',(11.0238490761438,0.,0.));
#4995=CARTESIAN_POINT('Origin',(16.3019119808107,0.,0.));
#4996=CARTESIAN_POINT('',(20.6781947947292,-9.21317321690256E-16,7.52312685038423));
#4997=CARTESIAN_POINT('Origin',(20.6781947947292,0.,0.));
#4998=CARTESIAN_POINT('',(16.3019119808107,-9.21317321690256E-16,7.52312685038423));
#4999=CARTESIAN_POINT('Origin',(20.9315098273138,0.,0.));
#5000=CARTESIAN_POINT('',(21.1848248598985,-8.82659349137786E-16,7.20746054905241));
#5001=CARTESIAN_POINT('',(20.9315098273138,9.01988335414021E-16,7.36529369971832));
#5002=CARTESIAN_POINT('Origin',(21.1848248598985,0.,0.));
#5003=CARTESIAN_POINT('Origin',(21.4140009475395,0.,0.));
#5004=CARTESIAN_POINT('',(21.6431770351805,-9.21957102532866E-16,7.52835105742136));
#5005=CARTESIAN_POINT('Origin',(21.6431770351805,0.,0.));
#5006=CARTESIAN_POINT('',(21.4140009475395,-9.02308225835327E-16,7.36790580323689));
#5007=CARTESIAN_POINT('Origin',(48.2427605064424,0.,0.));
#5008=CARTESIAN_POINT('',(74.8423439777042,-9.21957102532866E-16,7.52835105742136));
#5009=CARTESIAN_POINT('Origin',(74.8423439777042,0.,0.));
#5010=CARTESIAN_POINT('',(48.2427605064424,-9.21957102532866E-16,7.52835105742136));
#5011=CARTESIAN_POINT('Origin',(75.5565470559241,0.,0.));
#5012=CARTESIAN_POINT('',(76.270750134144,-7.86576021887409E-16,6.42288064146376));
#5013=CARTESIAN_POINT('',(75.5565470559241,8.54266562210138E-16,6.97561584944256));
#5014=CARTESIAN_POINT('Origin',(76.270750134144,0.,0.));
#5015=CARTESIAN_POINT('Origin',(53.9616500647475,0.,0.));
#5016=CARTESIAN_POINT('',(31.6525499953511,-7.84960767273423E-16,6.40969108660508));
#5017=CARTESIAN_POINT('Origin',(31.6525499953511,0.,0.));
#5018=CARTESIAN_POINT('',(53.9616500647475,-7.85768394580416E-16,6.41628586403442));
#5019=CARTESIAN_POINT('Origin',(31.0318089645314,0.,0.));
#5020=CARTESIAN_POINT('',(30.4110679337117,-7.84960767273423E-16,6.40969108660508));
#5021=CARTESIAN_POINT('Origin',(30.4110679337117,0.,0.));
#5022=CARTESIAN_POINT('',(31.0318089645314,-7.84960767273423E-16,6.40969108660508));
#5023=CARTESIAN_POINT('Origin',(29.5420239984498,0.,0.));
#5024=CARTESIAN_POINT('',(28.6729800631879,-7.84852901782084E-16,6.40881029802658));
#5025=CARTESIAN_POINT('Origin',(28.6729800631879,0.,0.));
#5026=CARTESIAN_POINT('',(29.5420239984498,-7.84884362648318E-16,6.40906719549494));
#5027=CARTESIAN_POINT('Origin',(28.6729800631879,0.,-6.41550316824698));
#5028=CARTESIAN_POINT('',(28.6729800631879,-7.85672541991337E-16,6.41550316824698));
#5029=CARTESIAN_POINT('Origin',(28.6729800631879,0.,0.));
#5030=CARTESIAN_POINT('Origin',(28.2136282688352,0.,0.));
#5031=CARTESIAN_POINT('',(27.7542764744824,-7.85672541991337E-16,6.41550316824698));
#5032=CARTESIAN_POINT('Origin',(27.7542764744824,0.,0.));
#5033=CARTESIAN_POINT('',(28.2136282688352,-7.85672541991337E-16,6.41550316824698));
#5034=CARTESIAN_POINT('Origin',(27.7542764744824,0.,-6.40853872070288));
#5035=CARTESIAN_POINT('',(27.7542764744824,-7.84819643152065E-16,6.40853872070288));
#5036=CARTESIAN_POINT('Origin',(27.7542764744824,0.,0.));
#5037=CARTESIAN_POINT('Origin',(26.6245076505395,0.,0.));
#5038=CARTESIAN_POINT('',(25.4947388265965,-7.84737844052149E-16,6.40787078036307));
#5039=CARTESIAN_POINT('Origin',(25.4947388265965,0.,0.));
#5040=CARTESIAN_POINT('',(26.6245076505395,-7.84778743602106E-16,6.40820475053297));
#5041=CARTESIAN_POINT('Origin',(25.0105689136245,0.,0.));
#5042=CARTESIAN_POINT('',(24.5263990006525,-7.84737844052149E-16,6.40787078036307));
#5043=CARTESIAN_POINT('Origin',(24.5263990006525,0.,0.));
#5044=CARTESIAN_POINT('',(25.0105689136245,-7.84737844052149E-16,6.40787078036307));
#5045=CARTESIAN_POINT('Origin',(23.6497386319918,0.,0.));
#5046=CARTESIAN_POINT('',(22.7730782633312,-7.84639315317936E-16,6.40706623219228));
#5047=CARTESIAN_POINT('Origin',(22.7730782633312,0.,0.));
#5048=CARTESIAN_POINT('',(23.6497386319918,-7.84671051911994E-16,6.40732538114918));
#5049=CARTESIAN_POINT('Origin',(22.2310089528171,0.,0.));
#5050=CARTESIAN_POINT('',(21.688939642303,-7.84639315317937E-16,6.40706623219228));
#5051=CARTESIAN_POINT('Origin',(21.688939642303,0.,0.));
#5052=CARTESIAN_POINT('',(22.2310089528171,-7.84639315317937E-16,6.40706623219228));
#5053=CARTESIAN_POINT('Origin',(21.4368822511007,0.,0.));
#5054=CARTESIAN_POINT('',(21.1848248598985,-7.8458181784762E-16,6.4065967297173));
#5055=CARTESIAN_POINT('Origin',(21.1848248598985,0.,0.));
#5056=CARTESIAN_POINT('',(21.4368822511007,-7.84590942753216E-16,6.40667124022599));
#5057=CARTESIAN_POINT('Origin',(21.1848248598985,0.,-4.66385643997278));
#5058=CARTESIAN_POINT('',(21.1848248598985,-5.71157686089543E-16,4.66385643997278));
#5059=CARTESIAN_POINT('Origin',(21.1848248598985,0.,0.));
#5060=CARTESIAN_POINT('Origin',(20.4983944566926,0.,0.));
#5061=CARTESIAN_POINT('',(19.8119640534868,-5.71157686089543E-16,4.66385643997278));
#5062=CARTESIAN_POINT('Origin',(19.8119640534868,0.,0.));
#5063=CARTESIAN_POINT('',(20.4983944566926,-5.71157686089543E-16,4.66385643997278));
#5064=CARTESIAN_POINT('Origin',(19.8119640534868,0.,-3.44589712386029));
#5065=CARTESIAN_POINT('',(19.8119640534868,-4.22000688292658E-16,3.44589712386029));
#5066=CARTESIAN_POINT('Origin',(19.8119640534868,0.,0.));
#5067=CARTESIAN_POINT('Origin',(15.9443326090014,0.,0.));
#5068=CARTESIAN_POINT('',(15.9443326090014,-4.22000688292657E-16,3.44589712386029));
#5069=CARTESIAN_POINT('Origin',(11.0238490761438,0.,-6.89179424772059));
#28033=UNCERTAINTY_MEASURE_WITH_UNIT(LENGTH_MEASURE(0.01),#28056,
'DISTANCE_ACCURACY_VALUE',
'Maximum model space distance between geometric entities at asserted c
onnectivities');
#28043=UNCERTAINTY_MEASURE_WITH_UNIT(LENGTH_MEASURE(0.01),#28056,
'DISTANCE_ACCURACY_VALUE',
'Maximum model space distance between geometric entities at asserted c
onnectivities');
#28045=(
GEOMETRIC_REPRESENTATION_CONTEXT(3)
GLOBAL_UNCERTAINTY_ASSIGNED_CONTEXT((#28033))
GLOBAL_UNIT_ASSIGNED_CONTEXT((#28056,#28058,#28059))
REPRESENTATION_CONTEXT('','3D')
);
#28055=(
GEOMETRIC_REPRESENTATION_CONTEXT(3)
GLOBAL_UNCERTAINTY_ASSIGNED_CONTEXT((#28043))
GLOBAL_UNIT_ASSIGNED_CONTEXT((#28056,#28058,#28059))
REPRESENTATION_CONTEXT('','3D')
);
#28056=(
LENGTH_UNIT()
NAMED_UNIT(*)
SI_UNIT(.MILLI.,.METRE.)
);
#28058=(
NAMED_UNIT(*)
PLANE_ANGLE_UNIT()
SI_UNIT($,.RADIAN.)
);
#28059=(
NAMED_UNIT(*)
SI_UNIT($,.STERADIAN.)
SOLID_ANGLE_UNIT()
);
#28061=SHAPE_DEFINITION_REPRESENTATION(#28072,#28093);
#28072=PRODUCT_DEFINITION_SHAPE('',$,#28105);
#28093=SHAPE_REPRESENTATION('',(#3801),#28045);
#28103=PRODUCT_DEFINITION_CONTEXT('part definition',#28138,'design');
#28105=PRODUCT_DEFINITION('Cylinder','Cylinder',#28116,#28103);
#28116=PRODUCT_DEFINITION_FORMATION('',$,#28141);
#28138=APPLICATION_CONTEXT(
'Core Data for Automotive Mechanical Design Process');
#28139=PRODUCT_CONTEXT('part definition',#28138,'mechanical');
#28141=PRODUCT('Cylinder','Cylinder',$,(#28139));
#28152=PRESENTATION_STYLE_ASSIGNMENT((#28155));
#28155=SURFACE_STYLE_USAGE(.BOTH.,#28158);
#28158=SURFACE_SIDE_STYLE('',(#28161));
#28161=SURFACE_STYLE_FILL_AREA(#28164);
#28164=FILL_AREA_STYLE('Opaque(160,160,160)',(#28167));
#28167=FILL_AREA_STYLE_COLOUR('Opaque(160,160,160)',#28170);
#28170=COLOUR_RGB('Opaque(160,160,160)', 0.66274510, 0.83137255, 0.94901961);
ENDSEC;
END-ISO-10303-21;
